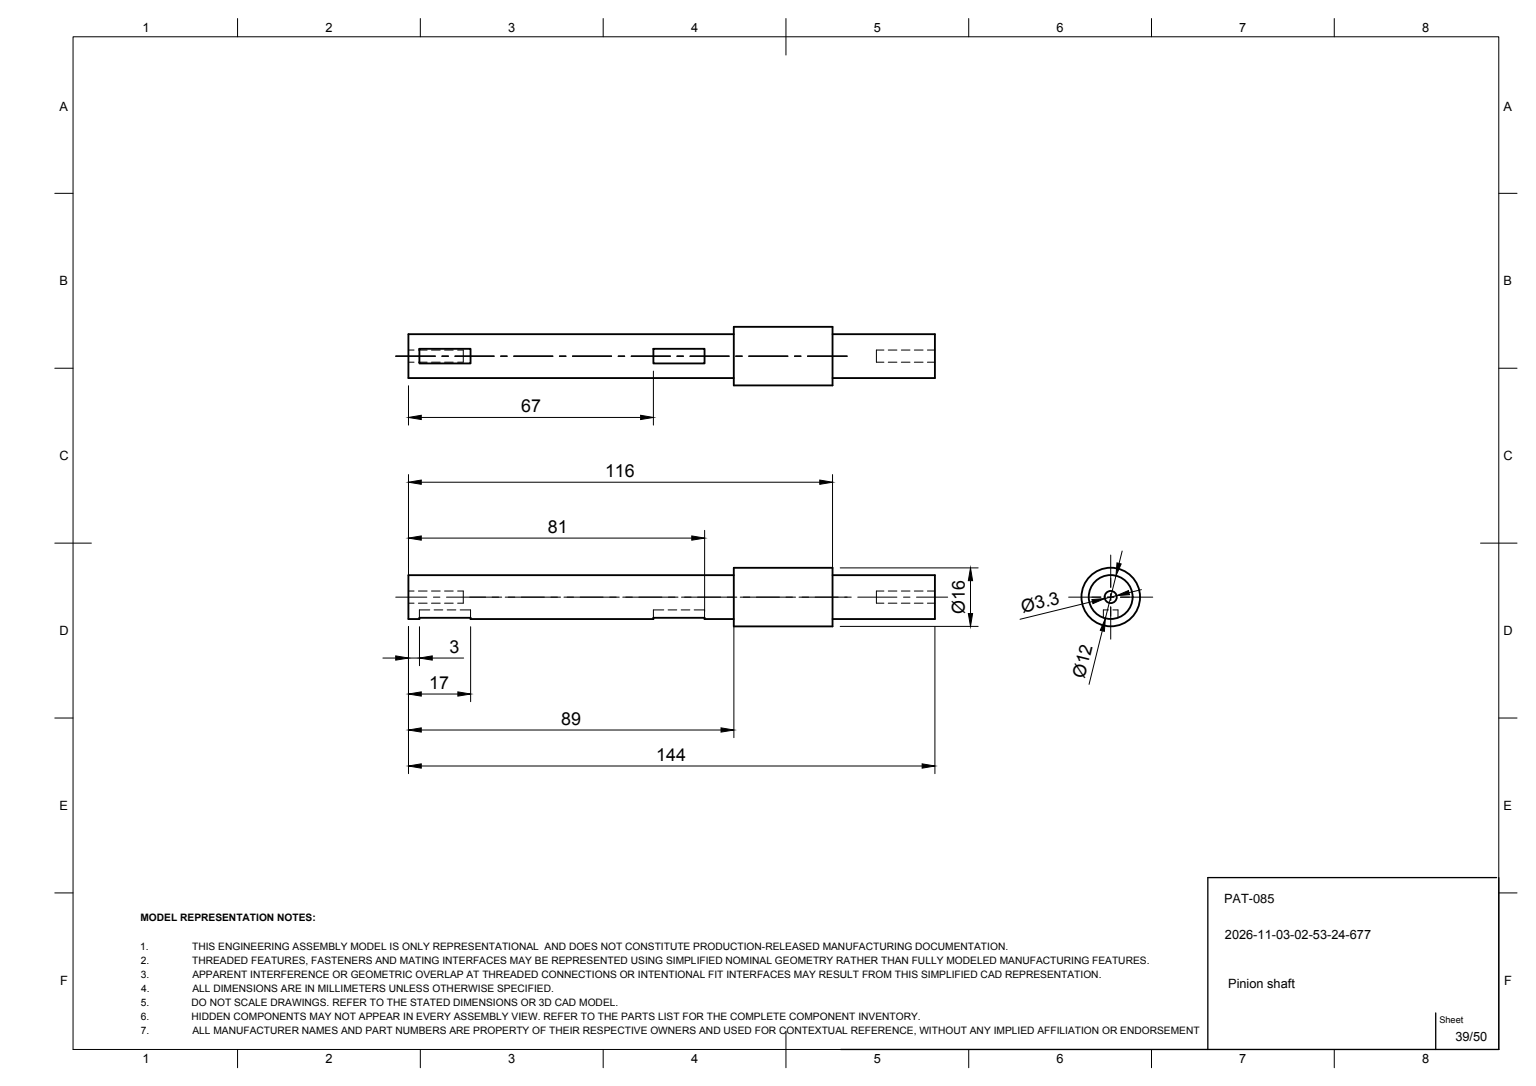
ISO-10303-21;
HEADER;
/* Generated by software containing ST-Developer
 * from STEP Tools, Inc. (www.steptools.com) 
 */

FILE_DESCRIPTION(
/* description */ ('Rack and pinion manual slide'),
/* implementation_level */ '2;1');

FILE_NAME(
/* name */ 'Pinion shaft.step',
/* time_stamp */ '2026-10-28T03:22:49-07:00',
/* author */ (''),
/* organization */ (''),
/* preprocessor_version */ 'ST-DEVELOPER v20.2',
/* originating_system */ 'Autodesk Translation Framework v15.17.0.0',
/* authorisation */ '');

FILE_SCHEMA (('AUTOMOTIVE_DESIGN { 1 0 10303 214 3 1 1 }'));
ENDSEC;

DATA;
#10=MECHANICAL_DESIGN_GEOMETRIC_PRESENTATION_REPRESENTATION('',(#770),#34851);
#671=SHAPE_REPRESENTATION_RELATIONSHIP('SRR','None',#35110,#717);
#717=ADVANCED_BREP_SHAPE_REPRESENTATION('',(#820),#34835);
#770=STYLED_ITEM('',(#35411),#820);
#820=MANIFOLD_SOLID_BREP('Body1',#13793);
#1010=FACE_BOUND('',#3003,.T.);
#1011=FACE_BOUND('',#3005,.T.);
#1012=FACE_BOUND('',#3009,.T.);
#1013=FACE_BOUND('',#3010,.T.);
#1014=FACE_BOUND('',#3012,.T.);
#1015=FACE_BOUND('',#3014,.T.);
#1434=PLANE('',#15200);
#1435=PLANE('',#15201);
#1436=PLANE('',#15203);
#1437=PLANE('',#15204);
#1438=PLANE('',#15205);
#1439=PLANE('',#15210);
#1440=PLANE('',#15214);
#1441=PLANE('',#15215);
#1442=PLANE('',#15216);
#1443=PLANE('',#15218);
#1444=PLANE('',#15219);
#1445=PLANE('',#15220);
#1446=PLANE('',#15222);
#1447=PLANE('',#15225);
#1448=PLANE('',#15233);
#1449=PLANE('',#15234);
#2072=FACE_OUTER_BOUND('',#2988,.T.);
#2073=FACE_OUTER_BOUND('',#2989,.T.);
#2074=FACE_OUTER_BOUND('',#2990,.T.);
#2075=FACE_OUTER_BOUND('',#2991,.T.);
#2076=FACE_OUTER_BOUND('',#2992,.T.);
#2077=FACE_OUTER_BOUND('',#2993,.T.);
#2078=FACE_OUTER_BOUND('',#2994,.T.);
#2079=FACE_OUTER_BOUND('',#2995,.T.);
#2080=FACE_OUTER_BOUND('',#2996,.T.);
#2081=FACE_OUTER_BOUND('',#2997,.T.);
#2082=FACE_OUTER_BOUND('',#2998,.T.);
#2083=FACE_OUTER_BOUND('',#2999,.T.);
#2084=FACE_OUTER_BOUND('',#3000,.T.);
#2085=FACE_OUTER_BOUND('',#3001,.T.);
#2086=FACE_OUTER_BOUND('',#3002,.T.);
#2087=FACE_OUTER_BOUND('',#3004,.T.);
#2088=FACE_OUTER_BOUND('',#3006,.T.);
#2089=FACE_OUTER_BOUND('',#3007,.T.);
#2090=FACE_OUTER_BOUND('',#3008,.T.);
#2091=FACE_OUTER_BOUND('',#3011,.T.);
#2092=FACE_OUTER_BOUND('',#3013,.T.);
#2988=EDGE_LOOP('',(#11912,#11913,#11914,#11915));
#2989=EDGE_LOOP('',(#11916,#11917,#11918,#11919));
#2990=EDGE_LOOP('',(#11920,#11921,#11922,#11923));
#2991=EDGE_LOOP('',(#11924,#11925,#11926,#11927));
#2992=EDGE_LOOP('',(#11928,#11929,#11930,#11931));
#2993=EDGE_LOOP('',(#11932,#11933,#11934,#11935));
#2994=EDGE_LOOP('',(#11936));
#2995=EDGE_LOOP('',(#11937,#11938,#11939,#11940));
#2996=EDGE_LOOP('',(#11941));
#2997=EDGE_LOOP('',(#11942,#11943,#11944,#11945));
#2998=EDGE_LOOP('',(#11946,#11947,#11948,#11949));
#2999=EDGE_LOOP('',(#11950,#11951,#11952,#11953));
#3000=EDGE_LOOP('',(#11954,#11955,#11956,#11957));
#3001=EDGE_LOOP('',(#11958,#11959,#11960,#11961));
#3002=EDGE_LOOP('',(#11962));
#3003=EDGE_LOOP('',(#11963));
#3004=EDGE_LOOP('',(#11964));
#3005=EDGE_LOOP('',(#11965));
#3006=EDGE_LOOP('',(#11966,#11967,#11968,#11969));
#3007=EDGE_LOOP('',(#11970,#11971,#11972,#11973));
#3008=EDGE_LOOP('',(#11974,#11975,#11976,#11977));
#3009=EDGE_LOOP('',(#11978,#11979,#11980,#11981));
#3010=EDGE_LOOP('',(#11982,#11983,#11984,#11985));
#3011=EDGE_LOOP('',(#11986));
#3012=EDGE_LOOP('',(#11987));
#3013=EDGE_LOOP('',(#11988));
#3014=EDGE_LOOP('',(#11989));
#4249=LINE('',#22573,#5540);
#4250=LINE('',#22575,#5541);
#4251=LINE('',#22577,#5542);
#4252=LINE('',#22578,#5543);
#4253=LINE('',#22583,#5544);
#4254=LINE('',#22584,#5545);
#4255=LINE('',#22587,#5546);
#4256=LINE('',#22589,#5547);
#4257=LINE('',#22590,#5548);
#4258=LINE('',#22592,#5549);
#4259=LINE('',#22599,#5550);
#4260=LINE('',#22606,#5551);
#4261=LINE('',#22612,#5552);
#4262=LINE('',#22614,#5553);
#4263=LINE('',#22616,#5554);
#4264=LINE('',#22617,#5555);
#4265=LINE('',#22622,#5556);
#4266=LINE('',#22623,#5557);
#4267=LINE('',#22626,#5558);
#4268=LINE('',#22628,#5559);
#4269=LINE('',#22629,#5560);
#4270=LINE('',#22631,#5561);
#4271=LINE('',#22645,#5562);
#4272=LINE('',#22648,#5563);
#4273=LINE('',#22653,#5564);
#5540=VECTOR('',#18393,1.);
#5541=VECTOR('',#18394,1.);
#5542=VECTOR('',#18395,1.);
#5543=VECTOR('',#18396,1.);
#5544=VECTOR('',#18401,1.);
#5545=VECTOR('',#18402,1.);
#5546=VECTOR('',#18405,1.);
#5547=VECTOR('',#18406,1.);
#5548=VECTOR('',#18407,1.);
#5549=VECTOR('',#18410,1.);
#5550=VECTOR('',#18419,0.164999999999999);
#5551=VECTOR('',#18428,0.164999999999999);
#5552=VECTOR('',#18435,1.);
#5553=VECTOR('',#18436,1.);
#5554=VECTOR('',#18437,1.);
#5555=VECTOR('',#18438,1.);
#5556=VECTOR('',#18443,1.);
#5557=VECTOR('',#18444,1.);
#5558=VECTOR('',#18447,1.);
#5559=VECTOR('',#18448,1.);
#5560=VECTOR('',#18449,1.);
#5561=VECTOR('',#18452,1.);
#5562=VECTOR('',#18471,0.800000000000001);
#5563=VECTOR('',#18474,0.6);
#5564=VECTOR('',#18481,0.6);
#6104=CIRCLE('',#15202,0.6);
#6105=CIRCLE('',#15206,0.6);
#6106=CIRCLE('',#15208,0.164999999999999);
#6107=CIRCLE('',#15209,0.164999999999999);
#6108=CIRCLE('',#15212,0.164999999999999);
#6109=CIRCLE('',#15213,0.164999999999999);
#6110=CIRCLE('',#15217,0.6);
#6111=CIRCLE('',#15221,0.6);
#6112=CIRCLE('',#15223,0.800000000000001);
#6113=CIRCLE('',#15224,0.6);
#6114=CIRCLE('',#15226,0.800000000000001);
#6115=CIRCLE('',#15227,0.6);
#6116=CIRCLE('',#15230,0.6);
#6117=CIRCLE('',#15232,0.6);
#7121=VERTEX_POINT('',#22571);
#7122=VERTEX_POINT('',#22572);
#7123=VERTEX_POINT('',#22574);
#7124=VERTEX_POINT('',#22576);
#7125=VERTEX_POINT('',#22580);
#7126=VERTEX_POINT('',#22582);
#7127=VERTEX_POINT('',#22586);
#7128=VERTEX_POINT('',#22588);
#7129=VERTEX_POINT('',#22596);
#7130=VERTEX_POINT('',#22598);
#7131=VERTEX_POINT('',#22603);
#7132=VERTEX_POINT('',#22605);
#7133=VERTEX_POINT('',#22610);
#7134=VERTEX_POINT('',#22611);
#7135=VERTEX_POINT('',#22613);
#7136=VERTEX_POINT('',#22615);
#7137=VERTEX_POINT('',#22619);
#7138=VERTEX_POINT('',#22621);
#7139=VERTEX_POINT('',#22625);
#7140=VERTEX_POINT('',#22627);
#7141=VERTEX_POINT('',#22635);
#7142=VERTEX_POINT('',#22637);
#7143=VERTEX_POINT('',#22640);
#7144=VERTEX_POINT('',#22642);
#7145=VERTEX_POINT('',#22647);
#7146=VERTEX_POINT('',#22651);
#8768=EDGE_CURVE('',#7121,#7122,#4249,.T.);
#8769=EDGE_CURVE('',#7121,#7123,#4250,.T.);
#8770=EDGE_CURVE('',#7124,#7123,#4251,.T.);
#8771=EDGE_CURVE('',#7124,#7122,#4252,.T.);
#8772=EDGE_CURVE('',#7122,#7125,#6104,.T.);
#8773=EDGE_CURVE('',#7126,#7124,#4253,.T.);
#8774=EDGE_CURVE('',#7125,#7126,#4254,.T.);
#8775=EDGE_CURVE('',#7125,#7127,#4255,.T.);
#8776=EDGE_CURVE('',#7126,#7128,#4256,.T.);
#8777=EDGE_CURVE('',#7128,#7127,#4257,.T.);
#8778=EDGE_CURVE('',#7123,#7128,#4258,.T.);
#8779=EDGE_CURVE('',#7127,#7121,#6105,.T.);
#8780=EDGE_CURVE('',#7129,#7129,#6106,.T.);
#8781=EDGE_CURVE('',#7129,#7130,#4259,.T.);
#8782=EDGE_CURVE('',#7130,#7130,#6107,.T.);
#8783=EDGE_CURVE('',#7131,#7131,#6108,.T.);
#8784=EDGE_CURVE('',#7131,#7132,#4260,.T.);
#8785=EDGE_CURVE('',#7132,#7132,#6109,.T.);
#8786=EDGE_CURVE('',#7133,#7134,#4261,.T.);
#8787=EDGE_CURVE('',#7133,#7135,#4262,.T.);
#8788=EDGE_CURVE('',#7136,#7135,#4263,.T.);
#8789=EDGE_CURVE('',#7136,#7134,#4264,.T.);
#8790=EDGE_CURVE('',#7134,#7137,#6110,.T.);
#8791=EDGE_CURVE('',#7138,#7136,#4265,.T.);
#8792=EDGE_CURVE('',#7137,#7138,#4266,.T.);
#8793=EDGE_CURVE('',#7137,#7139,#4267,.T.);
#8794=EDGE_CURVE('',#7138,#7140,#4268,.T.);
#8795=EDGE_CURVE('',#7140,#7139,#4269,.T.);
#8796=EDGE_CURVE('',#7135,#7140,#4270,.T.);
#8797=EDGE_CURVE('',#7139,#7133,#6111,.T.);
#8798=EDGE_CURVE('',#7141,#7141,#6112,.T.);
#8799=EDGE_CURVE('',#7142,#7142,#6113,.T.);
#8800=EDGE_CURVE('',#7143,#7143,#6114,.T.);
#8801=EDGE_CURVE('',#7144,#7144,#6115,.T.);
#8802=EDGE_CURVE('',#7141,#7143,#4271,.T.);
#8803=EDGE_CURVE('',#7144,#7145,#4272,.T.);
#8804=EDGE_CURVE('',#7145,#7145,#6116,.T.);
#8805=EDGE_CURVE('',#7146,#7146,#6117,.T.);
#8806=EDGE_CURVE('',#7146,#7142,#4273,.T.);
#11912=ORIENTED_EDGE('',*,*,#8768,.F.);
#11913=ORIENTED_EDGE('',*,*,#8769,.T.);
#11914=ORIENTED_EDGE('',*,*,#8770,.F.);
#11915=ORIENTED_EDGE('',*,*,#8771,.T.);
#11916=ORIENTED_EDGE('',*,*,#8772,.F.);
#11917=ORIENTED_EDGE('',*,*,#8771,.F.);
#11918=ORIENTED_EDGE('',*,*,#8773,.F.);
#11919=ORIENTED_EDGE('',*,*,#8774,.F.);
#11920=ORIENTED_EDGE('',*,*,#8775,.F.);
#11921=ORIENTED_EDGE('',*,*,#8774,.T.);
#11922=ORIENTED_EDGE('',*,*,#8776,.T.);
#11923=ORIENTED_EDGE('',*,*,#8777,.T.);
#11924=ORIENTED_EDGE('',*,*,#8773,.T.);
#11925=ORIENTED_EDGE('',*,*,#8770,.T.);
#11926=ORIENTED_EDGE('',*,*,#8778,.T.);
#11927=ORIENTED_EDGE('',*,*,#8776,.F.);
#11928=ORIENTED_EDGE('',*,*,#8779,.F.);
#11929=ORIENTED_EDGE('',*,*,#8777,.F.);
#11930=ORIENTED_EDGE('',*,*,#8778,.F.);
#11931=ORIENTED_EDGE('',*,*,#8769,.F.);
#11932=ORIENTED_EDGE('',*,*,#8780,.F.);
#11933=ORIENTED_EDGE('',*,*,#8781,.T.);
#11934=ORIENTED_EDGE('',*,*,#8782,.F.);
#11935=ORIENTED_EDGE('',*,*,#8781,.F.);
#11936=ORIENTED_EDGE('',*,*,#8780,.T.);
#11937=ORIENTED_EDGE('',*,*,#8783,.F.);
#11938=ORIENTED_EDGE('',*,*,#8784,.T.);
#11939=ORIENTED_EDGE('',*,*,#8785,.T.);
#11940=ORIENTED_EDGE('',*,*,#8784,.F.);
#11941=ORIENTED_EDGE('',*,*,#8785,.F.);
#11942=ORIENTED_EDGE('',*,*,#8786,.F.);
#11943=ORIENTED_EDGE('',*,*,#8787,.T.);
#11944=ORIENTED_EDGE('',*,*,#8788,.F.);
#11945=ORIENTED_EDGE('',*,*,#8789,.T.);
#11946=ORIENTED_EDGE('',*,*,#8790,.F.);
#11947=ORIENTED_EDGE('',*,*,#8789,.F.);
#11948=ORIENTED_EDGE('',*,*,#8791,.F.);
#11949=ORIENTED_EDGE('',*,*,#8792,.F.);
#11950=ORIENTED_EDGE('',*,*,#8793,.F.);
#11951=ORIENTED_EDGE('',*,*,#8792,.T.);
#11952=ORIENTED_EDGE('',*,*,#8794,.T.);
#11953=ORIENTED_EDGE('',*,*,#8795,.T.);
#11954=ORIENTED_EDGE('',*,*,#8791,.T.);
#11955=ORIENTED_EDGE('',*,*,#8788,.T.);
#11956=ORIENTED_EDGE('',*,*,#8796,.T.);
#11957=ORIENTED_EDGE('',*,*,#8794,.F.);
#11958=ORIENTED_EDGE('',*,*,#8797,.F.);
#11959=ORIENTED_EDGE('',*,*,#8795,.F.);
#11960=ORIENTED_EDGE('',*,*,#8796,.F.);
#11961=ORIENTED_EDGE('',*,*,#8787,.F.);
#11962=ORIENTED_EDGE('',*,*,#8798,.T.);
#11963=ORIENTED_EDGE('',*,*,#8799,.F.);
#11964=ORIENTED_EDGE('',*,*,#8800,.F.);
#11965=ORIENTED_EDGE('',*,*,#8801,.F.);
#11966=ORIENTED_EDGE('',*,*,#8798,.F.);
#11967=ORIENTED_EDGE('',*,*,#8802,.T.);
#11968=ORIENTED_EDGE('',*,*,#8800,.T.);
#11969=ORIENTED_EDGE('',*,*,#8802,.F.);
#11970=ORIENTED_EDGE('',*,*,#8801,.T.);
#11971=ORIENTED_EDGE('',*,*,#8803,.T.);
#11972=ORIENTED_EDGE('',*,*,#8804,.T.);
#11973=ORIENTED_EDGE('',*,*,#8803,.F.);
#11974=ORIENTED_EDGE('',*,*,#8805,.F.);
#11975=ORIENTED_EDGE('',*,*,#8806,.T.);
#11976=ORIENTED_EDGE('',*,*,#8799,.T.);
#11977=ORIENTED_EDGE('',*,*,#8806,.F.);
#11978=ORIENTED_EDGE('',*,*,#8775,.T.);
#11979=ORIENTED_EDGE('',*,*,#8779,.T.);
#11980=ORIENTED_EDGE('',*,*,#8768,.T.);
#11981=ORIENTED_EDGE('',*,*,#8772,.T.);
#11982=ORIENTED_EDGE('',*,*,#8793,.T.);
#11983=ORIENTED_EDGE('',*,*,#8797,.T.);
#11984=ORIENTED_EDGE('',*,*,#8786,.T.);
#11985=ORIENTED_EDGE('',*,*,#8790,.T.);
#11986=ORIENTED_EDGE('',*,*,#8805,.T.);
#11987=ORIENTED_EDGE('',*,*,#8782,.T.);
#11988=ORIENTED_EDGE('',*,*,#8804,.F.);
#11989=ORIENTED_EDGE('',*,*,#8783,.T.);
#12960=CYLINDRICAL_SURFACE('',#15207,0.164999999999999);
#12961=CYLINDRICAL_SURFACE('',#15211,0.164999999999999);
#12962=CYLINDRICAL_SURFACE('',#15228,0.800000000000001);
#12963=CYLINDRICAL_SURFACE('',#15229,0.6);
#12964=CYLINDRICAL_SURFACE('',#15231,0.6);
#13550=ADVANCED_FACE('',(#2072),#1434,.F.);
#13551=ADVANCED_FACE('',(#2073),#1435,.T.);
#13552=ADVANCED_FACE('',(#2074),#1436,.F.);
#13553=ADVANCED_FACE('',(#2075),#1437,.F.);
#13554=ADVANCED_FACE('',(#2076),#1438,.F.);
#13555=ADVANCED_FACE('',(#2077),#12960,.F.);
#13556=ADVANCED_FACE('',(#2078),#1439,.T.);
#13557=ADVANCED_FACE('',(#2079),#12961,.F.);
#13558=ADVANCED_FACE('',(#2080),#1440,.F.);
#13559=ADVANCED_FACE('',(#2081),#1441,.F.);
#13560=ADVANCED_FACE('',(#2082),#1442,.T.);
#13561=ADVANCED_FACE('',(#2083),#1443,.F.);
#13562=ADVANCED_FACE('',(#2084),#1444,.F.);
#13563=ADVANCED_FACE('',(#2085),#1445,.F.);
#13564=ADVANCED_FACE('',(#2086,#1010),#1446,.T.);
#13565=ADVANCED_FACE('',(#2087,#1011),#1447,.F.);
#13566=ADVANCED_FACE('',(#2088),#12962,.T.);
#13567=ADVANCED_FACE('',(#2089),#12963,.T.);
#13568=ADVANCED_FACE('',(#2090,#1012,#1013),#12964,.T.);
#13569=ADVANCED_FACE('',(#2091,#1014),#1448,.T.);
#13570=ADVANCED_FACE('',(#2092,#1015),#1449,.F.);
#13793=CLOSED_SHELL('',(#13550,#13551,#13552,#13553,#13554,#13555,#13556,
#13557,#13558,#13559,#13560,#13561,#13562,#13563,#13564,#13565,#13566,#13567,
#13568,#13569,#13570));
#15199=AXIS2_PLACEMENT_3D('',#22569,#18389,#18390);
#15200=AXIS2_PLACEMENT_3D('',#22570,#18391,#18392);
#15201=AXIS2_PLACEMENT_3D('',#22579,#18397,#18398);
#15202=AXIS2_PLACEMENT_3D('',#22581,#18399,#18400);
#15203=AXIS2_PLACEMENT_3D('',#22585,#18403,#18404);
#15204=AXIS2_PLACEMENT_3D('',#22591,#18408,#18409);
#15205=AXIS2_PLACEMENT_3D('',#22593,#18411,#18412);
#15206=AXIS2_PLACEMENT_3D('',#22594,#18413,#18414);
#15207=AXIS2_PLACEMENT_3D('',#22595,#18415,#18416);
#15208=AXIS2_PLACEMENT_3D('',#22597,#18417,#18418);
#15209=AXIS2_PLACEMENT_3D('',#22600,#18420,#18421);
#15210=AXIS2_PLACEMENT_3D('',#22601,#18422,#18423);
#15211=AXIS2_PLACEMENT_3D('',#22602,#18424,#18425);
#15212=AXIS2_PLACEMENT_3D('',#22604,#18426,#18427);
#15213=AXIS2_PLACEMENT_3D('',#22607,#18429,#18430);
#15214=AXIS2_PLACEMENT_3D('',#22608,#18431,#18432);
#15215=AXIS2_PLACEMENT_3D('',#22609,#18433,#18434);
#15216=AXIS2_PLACEMENT_3D('',#22618,#18439,#18440);
#15217=AXIS2_PLACEMENT_3D('',#22620,#18441,#18442);
#15218=AXIS2_PLACEMENT_3D('',#22624,#18445,#18446);
#15219=AXIS2_PLACEMENT_3D('',#22630,#18450,#18451);
#15220=AXIS2_PLACEMENT_3D('',#22632,#18453,#18454);
#15221=AXIS2_PLACEMENT_3D('',#22633,#18455,#18456);
#15222=AXIS2_PLACEMENT_3D('',#22634,#18457,#18458);
#15223=AXIS2_PLACEMENT_3D('',#22636,#18459,#18460);
#15224=AXIS2_PLACEMENT_3D('',#22638,#18461,#18462);
#15225=AXIS2_PLACEMENT_3D('',#22639,#18463,#18464);
#15226=AXIS2_PLACEMENT_3D('',#22641,#18465,#18466);
#15227=AXIS2_PLACEMENT_3D('',#22643,#18467,#18468);
#15228=AXIS2_PLACEMENT_3D('',#22644,#18469,#18470);
#15229=AXIS2_PLACEMENT_3D('',#22646,#18472,#18473);
#15230=AXIS2_PLACEMENT_3D('',#22649,#18475,#18476);
#15231=AXIS2_PLACEMENT_3D('',#22650,#18477,#18478);
#15232=AXIS2_PLACEMENT_3D('',#22652,#18479,#18480);
#15233=AXIS2_PLACEMENT_3D('',#22654,#18482,#18483);
#15234=AXIS2_PLACEMENT_3D('',#22655,#18484,#18485);
#18389=DIRECTION('axis',(0.,0.,1.));
#18390=DIRECTION('refdir',(1.,0.,0.));
#18391=DIRECTION('center_axis',(-1.,0.,0.));
#18392=DIRECTION('ref_axis',(0.,0.,1.));
#18393=DIRECTION('',(0.,-1.,0.));
#18394=DIRECTION('',(0.,0.,1.));
#18395=DIRECTION('',(0.,1.,0.));
#18396=DIRECTION('',(0.,0.,-1.));
#18397=DIRECTION('center_axis',(0.,1.,0.));
#18398=DIRECTION('ref_axis',(1.,0.,0.));
#18399=DIRECTION('center_axis',(0.,-1.,0.));
#18400=DIRECTION('ref_axis',(1.,0.,0.));
#18401=DIRECTION('',(-1.,0.,0.));
#18402=DIRECTION('',(0.,0.,1.));
#18403=DIRECTION('center_axis',(1.,0.,0.));
#18404=DIRECTION('ref_axis',(0.,0.,-1.));
#18405=DIRECTION('',(0.,1.,0.));
#18406=DIRECTION('',(0.,1.,0.));
#18407=DIRECTION('',(0.,0.,-1.));
#18408=DIRECTION('center_axis',(0.,0.,1.));
#18409=DIRECTION('ref_axis',(1.,0.,0.));
#18410=DIRECTION('',(1.,0.,0.));
#18411=DIRECTION('center_axis',(0.,1.,0.));
#18412=DIRECTION('ref_axis',(0.,0.,1.));
#18413=DIRECTION('center_axis',(0.,1.,0.));
#18414=DIRECTION('ref_axis',(1.,0.,0.));
#18415=DIRECTION('center_axis',(0.,1.,0.));
#18416=DIRECTION('ref_axis',(1.,0.,0.));
#18417=DIRECTION('center_axis',(0.,1.,0.));
#18418=DIRECTION('ref_axis',(1.,0.,0.));
#18419=DIRECTION('',(0.,1.,0.));
#18420=DIRECTION('center_axis',(0.,-1.,0.));
#18421=DIRECTION('ref_axis',(1.,0.,0.));
#18422=DIRECTION('center_axis',(0.,1.,0.));
#18423=DIRECTION('ref_axis',(1.,0.,0.));
#18424=DIRECTION('center_axis',(0.,1.,0.));
#18425=DIRECTION('ref_axis',(1.,0.,0.));
#18426=DIRECTION('center_axis',(0.,1.,0.));
#18427=DIRECTION('ref_axis',(1.,0.,0.));
#18428=DIRECTION('',(0.,1.,0.));
#18429=DIRECTION('center_axis',(0.,1.,0.));
#18430=DIRECTION('ref_axis',(1.,0.,0.));
#18431=DIRECTION('center_axis',(0.,1.,0.));
#18432=DIRECTION('ref_axis',(1.,0.,0.));
#18433=DIRECTION('center_axis',(-1.,0.,0.));
#18434=DIRECTION('ref_axis',(0.,0.,1.));
#18435=DIRECTION('',(0.,-1.,0.));
#18436=DIRECTION('',(0.,0.,1.));
#18437=DIRECTION('',(0.,1.,0.));
#18438=DIRECTION('',(0.,0.,-1.));
#18439=DIRECTION('center_axis',(0.,1.,0.));
#18440=DIRECTION('ref_axis',(1.,0.,0.));
#18441=DIRECTION('center_axis',(0.,-1.,0.));
#18442=DIRECTION('ref_axis',(1.,0.,0.));
#18443=DIRECTION('',(-1.,0.,0.));
#18444=DIRECTION('',(0.,0.,1.));
#18445=DIRECTION('center_axis',(1.,0.,0.));
#18446=DIRECTION('ref_axis',(0.,0.,-1.));
#18447=DIRECTION('',(0.,1.,0.));
#18448=DIRECTION('',(0.,1.,0.));
#18449=DIRECTION('',(0.,0.,-1.));
#18450=DIRECTION('center_axis',(0.,0.,1.));
#18451=DIRECTION('ref_axis',(1.,0.,0.));
#18452=DIRECTION('',(1.,0.,0.));
#18453=DIRECTION('center_axis',(0.,1.,0.));
#18454=DIRECTION('ref_axis',(0.,0.,1.));
#18455=DIRECTION('center_axis',(0.,1.,0.));
#18456=DIRECTION('ref_axis',(1.,0.,0.));
#18457=DIRECTION('center_axis',(0.,1.,0.));
#18458=DIRECTION('ref_axis',(1.,0.,0.));
#18459=DIRECTION('center_axis',(0.,1.,0.));
#18460=DIRECTION('ref_axis',(1.,0.,0.));
#18461=DIRECTION('center_axis',(0.,1.,0.));
#18462=DIRECTION('ref_axis',(1.,0.,0.));
#18463=DIRECTION('center_axis',(0.,1.,0.));
#18464=DIRECTION('ref_axis',(1.,0.,0.));
#18465=DIRECTION('center_axis',(0.,1.,0.));
#18466=DIRECTION('ref_axis',(1.,0.,0.));
#18467=DIRECTION('center_axis',(0.,-1.,0.));
#18468=DIRECTION('ref_axis',(1.,0.,0.));
#18469=DIRECTION('center_axis',(0.,1.,0.));
#18470=DIRECTION('ref_axis',(1.,0.,0.));
#18471=DIRECTION('',(0.,-1.,0.));
#18472=DIRECTION('center_axis',(0.,1.,0.));
#18473=DIRECTION('ref_axis',(1.,0.,0.));
#18474=DIRECTION('',(0.,-1.,0.));
#18475=DIRECTION('center_axis',(0.,1.,0.));
#18476=DIRECTION('ref_axis',(1.,0.,0.));
#18477=DIRECTION('center_axis',(0.,1.,0.));
#18478=DIRECTION('ref_axis',(1.,0.,0.));
#18479=DIRECTION('center_axis',(0.,1.,0.));
#18480=DIRECTION('ref_axis',(1.,0.,0.));
#18481=DIRECTION('',(0.,-1.,0.));
#18482=DIRECTION('center_axis',(0.,1.,0.));
#18483=DIRECTION('ref_axis',(1.,0.,0.));
#18484=DIRECTION('center_axis',(0.,1.,0.));
#18485=DIRECTION('ref_axis',(1.,0.,0.));
#22569=CARTESIAN_POINT('',(0.,0.,0.));
#22570=CARTESIAN_POINT('Origin',(10.8,6.2,9.55));
#22571=CARTESIAN_POINT('',(10.8,7.6,9.68431457505076));
#22572=CARTESIAN_POINT('',(10.8,6.2,9.68431457505076));
#22573=CARTESIAN_POINT('',(10.8,-6.5,9.68431457505076));
#22574=CARTESIAN_POINT('',(10.8,7.6,9.9));
#22575=CARTESIAN_POINT('',(10.8,7.6,9.9));
#22576=CARTESIAN_POINT('',(10.8,6.2,9.9));
#22577=CARTESIAN_POINT('',(10.8,6.2,9.9));
#22578=CARTESIAN_POINT('',(10.8,6.2,9.9));
#22579=CARTESIAN_POINT('Origin',(11.,6.2,9.725));
#22580=CARTESIAN_POINT('',(11.2,6.2,9.68431457505076));
#22581=CARTESIAN_POINT('Origin',(11.,6.2,10.25));
#22582=CARTESIAN_POINT('',(11.2,6.2,9.9));
#22583=CARTESIAN_POINT('',(11.2,6.2,9.9));
#22584=CARTESIAN_POINT('',(11.2,6.2,9.55));
#22585=CARTESIAN_POINT('Origin',(11.2,6.2,9.9));
#22586=CARTESIAN_POINT('',(11.2,7.6,9.68431457505076));
#22587=CARTESIAN_POINT('',(11.2,-6.5,9.68431457505076));
#22588=CARTESIAN_POINT('',(11.2,7.6,9.9));
#22589=CARTESIAN_POINT('',(11.2,6.2,9.9));
#22590=CARTESIAN_POINT('',(11.2,7.6,9.55));
#22591=CARTESIAN_POINT('Origin',(10.8,6.2,9.9));
#22592=CARTESIAN_POINT('',(11.2,7.6,9.9));
#22593=CARTESIAN_POINT('Origin',(11.,7.6,9.725));
#22594=CARTESIAN_POINT('Origin',(11.,7.6,10.25));
#22595=CARTESIAN_POINT('Origin',(11.,6.4,10.25));
#22596=CARTESIAN_POINT('',(10.835,6.4,10.25));
#22597=CARTESIAN_POINT('Origin',(11.,6.4,10.25));
#22598=CARTESIAN_POINT('',(10.835,7.9,10.25));
#22599=CARTESIAN_POINT('',(10.835,6.4,10.25));
#22600=CARTESIAN_POINT('Origin',(11.,7.9,10.25));
#22601=CARTESIAN_POINT('Origin',(11.,6.4,10.25));
#22602=CARTESIAN_POINT('Origin',(11.,-6.6,10.25));
#22603=CARTESIAN_POINT('',(10.835,-6.5,10.25));
#22604=CARTESIAN_POINT('Origin',(11.,-6.5,10.25));
#22605=CARTESIAN_POINT('',(10.835,-4.9,10.25));
#22606=CARTESIAN_POINT('',(10.835,-6.6,10.25));
#22607=CARTESIAN_POINT('Origin',(11.,-4.9,10.25));
#22608=CARTESIAN_POINT('Origin',(11.,-4.9,10.25));
#22609=CARTESIAN_POINT('Origin',(10.8,-0.2,9.55));
#22610=CARTESIAN_POINT('',(10.8,1.2,9.68431457505076));
#22611=CARTESIAN_POINT('',(10.8,-0.2,9.68431457505076));
#22612=CARTESIAN_POINT('',(10.8,-6.5,9.68431457505076));
#22613=CARTESIAN_POINT('',(10.8,1.2,9.9));
#22614=CARTESIAN_POINT('',(10.8,1.2,9.9));
#22615=CARTESIAN_POINT('',(10.8,-0.2,9.9));
#22616=CARTESIAN_POINT('',(10.8,-0.2,9.9));
#22617=CARTESIAN_POINT('',(10.8,-0.2,9.9));
#22618=CARTESIAN_POINT('Origin',(11.,-0.2,9.725));
#22619=CARTESIAN_POINT('',(11.2,-0.2,9.68431457505076));
#22620=CARTESIAN_POINT('Origin',(11.,-0.2,10.25));
#22621=CARTESIAN_POINT('',(11.2,-0.2,9.9));
#22622=CARTESIAN_POINT('',(11.2,-0.2,9.9));
#22623=CARTESIAN_POINT('',(11.2,-0.2,9.55));
#22624=CARTESIAN_POINT('Origin',(11.2,-0.2,9.9));
#22625=CARTESIAN_POINT('',(11.2,1.2,9.68431457505076));
#22626=CARTESIAN_POINT('',(11.2,-6.5,9.68431457505076));
#22627=CARTESIAN_POINT('',(11.2,1.2,9.9));
#22628=CARTESIAN_POINT('',(11.2,-0.2,9.9));
#22629=CARTESIAN_POINT('',(11.2,1.2,9.55));
#22630=CARTESIAN_POINT('Origin',(10.8,-0.2,9.9));
#22631=CARTESIAN_POINT('',(11.2,1.2,9.9));
#22632=CARTESIAN_POINT('Origin',(11.,1.2,9.725));
#22633=CARTESIAN_POINT('Origin',(11.,1.2,10.25));
#22634=CARTESIAN_POINT('Origin',(11.,-1.,10.25));
#22635=CARTESIAN_POINT('',(10.2,-1.,10.25));
#22636=CARTESIAN_POINT('Origin',(11.,-1.,10.25));
#22637=CARTESIAN_POINT('',(10.4,-1.,10.25));
#22638=CARTESIAN_POINT('Origin',(11.,-1.,10.25));
#22639=CARTESIAN_POINT('Origin',(11.,-3.7,10.25));
#22640=CARTESIAN_POINT('',(10.2,-3.7,10.25));
#22641=CARTESIAN_POINT('Origin',(11.,-3.7,10.25));
#22642=CARTESIAN_POINT('',(10.4,-3.7,10.25));
#22643=CARTESIAN_POINT('Origin',(11.,-3.7,10.25));
#22644=CARTESIAN_POINT('Origin',(11.,-3.7,10.25));
#22645=CARTESIAN_POINT('',(10.2,-3.7,10.25));
#22646=CARTESIAN_POINT('Origin',(11.,-6.5,10.25));
#22647=CARTESIAN_POINT('',(10.4,-6.5,10.25));
#22648=CARTESIAN_POINT('',(10.4,-6.5,10.25));
#22649=CARTESIAN_POINT('Origin',(11.,-6.5,10.25));
#22650=CARTESIAN_POINT('Origin',(11.,-6.5,10.25));
#22651=CARTESIAN_POINT('',(10.4,7.9,10.25));
#22652=CARTESIAN_POINT('Origin',(11.,7.9,10.25));
#22653=CARTESIAN_POINT('',(10.4,-6.5,10.25));
#22654=CARTESIAN_POINT('Origin',(11.,7.9,10.25));
#22655=CARTESIAN_POINT('Origin',(11.,-6.5,10.25));
#34781=UNCERTAINTY_MEASURE_WITH_UNIT(LENGTH_MEASURE(0.001),#34852,
'DISTANCE_ACCURACY_VALUE',
'Maximum model space distance between geometric entities at asserted c
onnectivities');
#34797=UNCERTAINTY_MEASURE_WITH_UNIT(LENGTH_MEASURE(0.001),#34852,
'DISTANCE_ACCURACY_VALUE',
'Maximum model space distance between geometric entities at asserted c
onnectivities');
#34835=(
GEOMETRIC_REPRESENTATION_CONTEXT(3)
GLOBAL_UNCERTAINTY_ASSIGNED_CONTEXT((#34781))
GLOBAL_UNIT_ASSIGNED_CONTEXT((#34852,#34854,#34855))
REPRESENTATION_CONTEXT('','3D')
);
#34851=(
GEOMETRIC_REPRESENTATION_CONTEXT(3)
GLOBAL_UNCERTAINTY_ASSIGNED_CONTEXT((#34797))
GLOBAL_UNIT_ASSIGNED_CONTEXT((#34852,#34854,#34855))
REPRESENTATION_CONTEXT('','3D')
);
#34852=(
LENGTH_UNIT()
NAMED_UNIT(*)
SI_UNIT(.CENTI.,.METRE.)
);
#34854=(
NAMED_UNIT(*)
PLANE_ANGLE_UNIT()
SI_UNIT($,.RADIAN.)
);
#34855=(
NAMED_UNIT(*)
SI_UNIT($,.STERADIAN.)
SOLID_ANGLE_UNIT()
);
#34893=SHAPE_DEFINITION_REPRESENTATION(#34954,#35110);
#34954=PRODUCT_DEFINITION_SHAPE('',$,#35164);
#35110=SHAPE_REPRESENTATION('',(#15199),#34835);
#35126=PRODUCT_DEFINITION_CONTEXT('part definition',#35287,'design');
#35164=PRODUCT_DEFINITION('Pinion shaft','Pinion shaft',#35217,#35126);
#35217=PRODUCT_DEFINITION_FORMATION('',$,#35326);
#35287=APPLICATION_CONTEXT(
'Core Data for Automotive Mechanical Design Process');
#35288=PRODUCT_CONTEXT('part definition',#35287,'mechanical');
#35326=PRODUCT('Pinion shaft','Pinion shaft','Pinion shaft',(#35288));
#35405=COLOUR_RGB('Grey',0.48,0.52,0.57);
#35406=FILL_AREA_STYLE_COLOUR('',#35405);
#35407=FILL_AREA_STYLE('',(#35406));
#35408=SURFACE_STYLE_FILL_AREA(#35407);
#35409=SURFACE_SIDE_STYLE('',(#35408));
#35410=SURFACE_STYLE_USAGE(.BOTH.,#35409);
#35411=PRESENTATION_STYLE_ASSIGNMENT((#35410));
ENDSEC;
END-ISO-10303-21;
